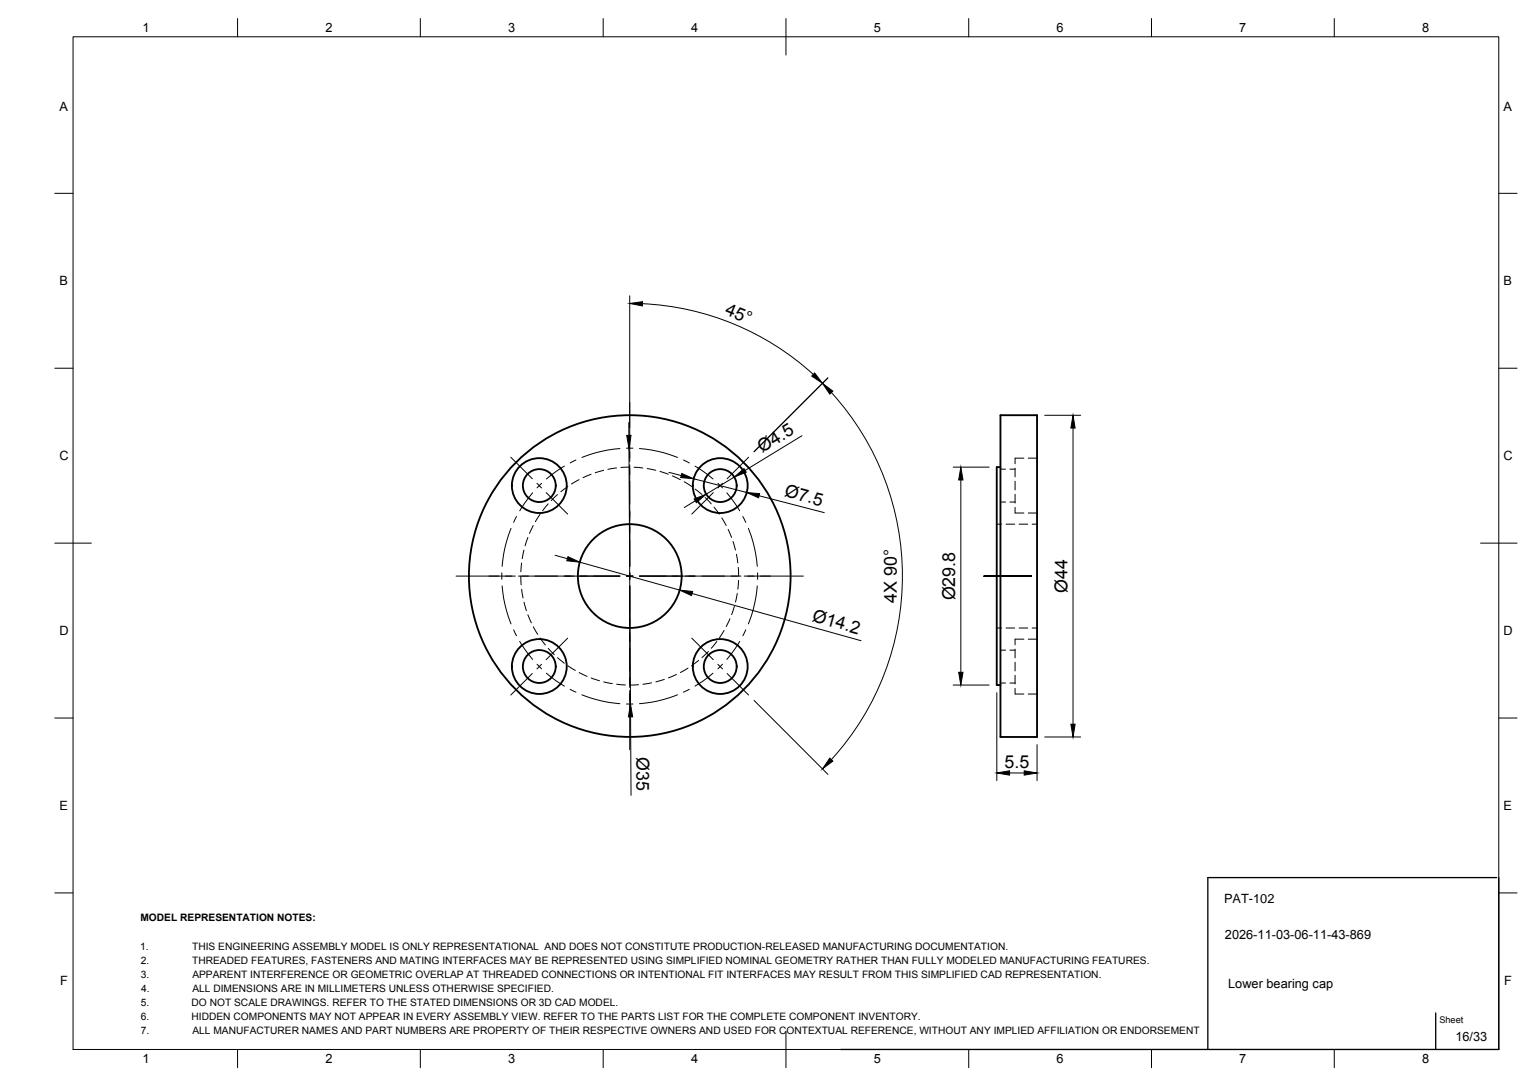
ISO-10303-21;
HEADER;
/* Generated by software containing ST-Developer
 * from STEP Tools, Inc. (www.steptools.com) 
 */

FILE_DESCRIPTION(
/* description */ ('Swing-away clamp arm'),
/* implementation_level */ '2;1');

FILE_NAME(
/* name */ 'Lower bearing cap.step',
/* time_stamp */ '2026-10-28T03:26:03-07:00',
/* author */ (''),
/* organization */ (''),
/* preprocessor_version */ 'ST-DEVELOPER v20.2',
/* originating_system */ 'Autodesk Translation Framework v15.17.0.0',
/* authorisation */ '');

FILE_SCHEMA (('AUTOMOTIVE_DESIGN { 1 0 10303 214 3 1 1 }'));
ENDSEC;

DATA;
#10=MECHANICAL_DESIGN_GEOMETRIC_PRESENTATION_REPRESENTATION('',(#303),#10627);
#251=SHAPE_REPRESENTATION_RELATIONSHIP('SRR','None',#10750,#277);
#277=ADVANCED_BREP_SHAPE_REPRESENTATION('',(#336),#10609);
#303=STYLED_ITEM('',(#10965),#336);
#336=MANIFOLD_SOLID_BREP('Body1',#4910);
#401=FACE_BOUND('',#1128,.T.);
#402=FACE_BOUND('',#1131,.T.);
#403=FACE_BOUND('',#1134,.T.);
#404=FACE_BOUND('',#1137,.T.);
#405=FACE_BOUND('',#1144,.T.);
#406=FACE_BOUND('',#1148,.T.);
#407=FACE_BOUND('',#1149,.T.);
#408=FACE_BOUND('',#1150,.T.);
#409=FACE_BOUND('',#1151,.T.);
#410=FACE_BOUND('',#1152,.T.);
#411=FACE_BOUND('',#1154,.T.);
#412=FACE_BOUND('',#1155,.T.);
#413=FACE_BOUND('',#1156,.T.);
#414=FACE_BOUND('',#1157,.T.);
#415=FACE_BOUND('',#1158,.T.);
#556=PLANE('',#5482);
#557=PLANE('',#5487);
#558=PLANE('',#5492);
#559=PLANE('',#5497);
#560=PLANE('',#5510);
#561=PLANE('',#5517);
#562=PLANE('',#5518);
#776=FACE_OUTER_BOUND('',#1126,.T.);
#777=FACE_OUTER_BOUND('',#1127,.T.);
#778=FACE_OUTER_BOUND('',#1129,.T.);
#779=FACE_OUTER_BOUND('',#1130,.T.);
#780=FACE_OUTER_BOUND('',#1132,.T.);
#781=FACE_OUTER_BOUND('',#1133,.T.);
#782=FACE_OUTER_BOUND('',#1135,.T.);
#783=FACE_OUTER_BOUND('',#1136,.T.);
#784=FACE_OUTER_BOUND('',#1138,.T.);
#785=FACE_OUTER_BOUND('',#1139,.T.);
#786=FACE_OUTER_BOUND('',#1140,.T.);
#787=FACE_OUTER_BOUND('',#1141,.T.);
#788=FACE_OUTER_BOUND('',#1142,.T.);
#789=FACE_OUTER_BOUND('',#1143,.T.);
#790=FACE_OUTER_BOUND('',#1145,.T.);
#791=FACE_OUTER_BOUND('',#1146,.T.);
#792=FACE_OUTER_BOUND('',#1147,.T.);
#793=FACE_OUTER_BOUND('',#1153,.T.);
#1126=EDGE_LOOP('',(#3873,#3874,#3875,#3876));
#1127=EDGE_LOOP('',(#3877));
#1128=EDGE_LOOP('',(#3878));
#1129=EDGE_LOOP('',(#3879,#3880,#3881,#3882));
#1130=EDGE_LOOP('',(#3883));
#1131=EDGE_LOOP('',(#3884));
#1132=EDGE_LOOP('',(#3885,#3886,#3887,#3888));
#1133=EDGE_LOOP('',(#3889));
#1134=EDGE_LOOP('',(#3890));
#1135=EDGE_LOOP('',(#3891,#3892,#3893,#3894));
#1136=EDGE_LOOP('',(#3895));
#1137=EDGE_LOOP('',(#3896));
#1138=EDGE_LOOP('',(#3897,#3898,#3899,#3900));
#1139=EDGE_LOOP('',(#3901,#3902,#3903,#3904));
#1140=EDGE_LOOP('',(#3905,#3906,#3907,#3908));
#1141=EDGE_LOOP('',(#3909,#3910,#3911,#3912));
#1142=EDGE_LOOP('',(#3913,#3914,#3915,#3916));
#1143=EDGE_LOOP('',(#3917));
#1144=EDGE_LOOP('',(#3918));
#1145=EDGE_LOOP('',(#3919,#3920,#3921,#3922));
#1146=EDGE_LOOP('',(#3923,#3924,#3925,#3926));
#1147=EDGE_LOOP('',(#3927));
#1148=EDGE_LOOP('',(#3928));
#1149=EDGE_LOOP('',(#3929));
#1150=EDGE_LOOP('',(#3930));
#1151=EDGE_LOOP('',(#3931));
#1152=EDGE_LOOP('',(#3932));
#1153=EDGE_LOOP('',(#3933));
#1154=EDGE_LOOP('',(#3934));
#1155=EDGE_LOOP('',(#3935));
#1156=EDGE_LOOP('',(#3936));
#1157=EDGE_LOOP('',(#3937));
#1158=EDGE_LOOP('',(#3938));
#1552=LINE('',#9485,#1874);
#1553=LINE('',#9494,#1875);
#1554=LINE('',#9503,#1876);
#1555=LINE('',#9512,#1877);
#1556=LINE('',#9519,#1878);
#1557=LINE('',#9523,#1879);
#1558=LINE('',#9527,#1880);
#1559=LINE('',#9531,#1881);
#1560=LINE('',#9537,#1882);
#1561=LINE('',#9544,#1883);
#1562=LINE('',#9550,#1884);
#1874=VECTOR('',#6587,0.375);
#1875=VECTOR('',#6598,0.375);
#1876=VECTOR('',#6609,0.375);
#1877=VECTOR('',#6620,0.375);
#1878=VECTOR('',#6629,0.225);
#1879=VECTOR('',#6634,0.225);
#1880=VECTOR('',#6639,0.225);
#1881=VECTOR('',#6644,0.225);
#1882=VECTOR('',#6651,1.49);
#1883=VECTOR('',#6660,0.71);
#1884=VECTOR('',#6667,2.2);
#2089=CIRCLE('',#5480,0.375);
#2090=CIRCLE('',#5481,0.375);
#2091=CIRCLE('',#5483,0.225);
#2092=CIRCLE('',#5485,0.375);
#2093=CIRCLE('',#5486,0.375);
#2094=CIRCLE('',#5488,0.225);
#2095=CIRCLE('',#5490,0.375);
#2096=CIRCLE('',#5491,0.375);
#2097=CIRCLE('',#5493,0.225);
#2098=CIRCLE('',#5495,0.375);
#2099=CIRCLE('',#5496,0.375);
#2100=CIRCLE('',#5498,0.225);
#2101=CIRCLE('',#5500,0.225);
#2102=CIRCLE('',#5502,0.225);
#2103=CIRCLE('',#5504,0.225);
#2104=CIRCLE('',#5506,0.225);
#2105=CIRCLE('',#5508,1.49);
#2106=CIRCLE('',#5509,1.49);
#2107=CIRCLE('',#5511,0.71);
#2108=CIRCLE('',#5513,0.71);
#2109=CIRCLE('',#5515,2.2);
#2110=CIRCLE('',#5516,2.2);
#2458=VERTEX_POINT('',#9482);
#2459=VERTEX_POINT('',#9484);
#2460=VERTEX_POINT('',#9488);
#2461=VERTEX_POINT('',#9491);
#2462=VERTEX_POINT('',#9493);
#2463=VERTEX_POINT('',#9497);
#2464=VERTEX_POINT('',#9500);
#2465=VERTEX_POINT('',#9502);
#2466=VERTEX_POINT('',#9506);
#2467=VERTEX_POINT('',#9509);
#2468=VERTEX_POINT('',#9511);
#2469=VERTEX_POINT('',#9515);
#2470=VERTEX_POINT('',#9518);
#2471=VERTEX_POINT('',#9522);
#2472=VERTEX_POINT('',#9526);
#2473=VERTEX_POINT('',#9530);
#2474=VERTEX_POINT('',#9534);
#2475=VERTEX_POINT('',#9536);
#2476=VERTEX_POINT('',#9540);
#2477=VERTEX_POINT('',#9543);
#2478=VERTEX_POINT('',#9547);
#2479=VERTEX_POINT('',#9549);
#2969=EDGE_CURVE('',#2458,#2458,#2089,.T.);
#2970=EDGE_CURVE('',#2458,#2459,#1552,.T.);
#2971=EDGE_CURVE('',#2459,#2459,#2090,.T.);
#2972=EDGE_CURVE('',#2460,#2460,#2091,.T.);
#2973=EDGE_CURVE('',#2461,#2461,#2092,.T.);
#2974=EDGE_CURVE('',#2461,#2462,#1553,.T.);
#2975=EDGE_CURVE('',#2462,#2462,#2093,.T.);
#2976=EDGE_CURVE('',#2463,#2463,#2094,.T.);
#2977=EDGE_CURVE('',#2464,#2464,#2095,.T.);
#2978=EDGE_CURVE('',#2464,#2465,#1554,.T.);
#2979=EDGE_CURVE('',#2465,#2465,#2096,.T.);
#2980=EDGE_CURVE('',#2466,#2466,#2097,.T.);
#2981=EDGE_CURVE('',#2467,#2467,#2098,.T.);
#2982=EDGE_CURVE('',#2467,#2468,#1555,.T.);
#2983=EDGE_CURVE('',#2468,#2468,#2099,.T.);
#2984=EDGE_CURVE('',#2469,#2469,#2100,.T.);
#2985=EDGE_CURVE('',#2460,#2470,#1556,.T.);
#2986=EDGE_CURVE('',#2470,#2470,#2101,.T.);
#2987=EDGE_CURVE('',#2463,#2471,#1557,.T.);
#2988=EDGE_CURVE('',#2471,#2471,#2102,.T.);
#2989=EDGE_CURVE('',#2466,#2472,#1558,.T.);
#2990=EDGE_CURVE('',#2472,#2472,#2103,.T.);
#2991=EDGE_CURVE('',#2469,#2473,#1559,.T.);
#2992=EDGE_CURVE('',#2473,#2473,#2104,.T.);
#2993=EDGE_CURVE('',#2474,#2474,#2105,.T.);
#2994=EDGE_CURVE('',#2474,#2475,#1560,.T.);
#2995=EDGE_CURVE('',#2475,#2475,#2106,.T.);
#2996=EDGE_CURVE('',#2476,#2476,#2107,.T.);
#2997=EDGE_CURVE('',#2476,#2477,#1561,.T.);
#2998=EDGE_CURVE('',#2477,#2477,#2108,.T.);
#2999=EDGE_CURVE('',#2478,#2478,#2109,.T.);
#3000=EDGE_CURVE('',#2478,#2479,#1562,.T.);
#3001=EDGE_CURVE('',#2479,#2479,#2110,.T.);
#3873=ORIENTED_EDGE('',*,*,#2969,.F.);
#3874=ORIENTED_EDGE('',*,*,#2970,.T.);
#3875=ORIENTED_EDGE('',*,*,#2971,.T.);
#3876=ORIENTED_EDGE('',*,*,#2970,.F.);
#3877=ORIENTED_EDGE('',*,*,#2971,.F.);
#3878=ORIENTED_EDGE('',*,*,#2972,.F.);
#3879=ORIENTED_EDGE('',*,*,#2973,.F.);
#3880=ORIENTED_EDGE('',*,*,#2974,.T.);
#3881=ORIENTED_EDGE('',*,*,#2975,.T.);
#3882=ORIENTED_EDGE('',*,*,#2974,.F.);
#3883=ORIENTED_EDGE('',*,*,#2975,.F.);
#3884=ORIENTED_EDGE('',*,*,#2976,.F.);
#3885=ORIENTED_EDGE('',*,*,#2977,.F.);
#3886=ORIENTED_EDGE('',*,*,#2978,.T.);
#3887=ORIENTED_EDGE('',*,*,#2979,.T.);
#3888=ORIENTED_EDGE('',*,*,#2978,.F.);
#3889=ORIENTED_EDGE('',*,*,#2979,.F.);
#3890=ORIENTED_EDGE('',*,*,#2980,.F.);
#3891=ORIENTED_EDGE('',*,*,#2981,.F.);
#3892=ORIENTED_EDGE('',*,*,#2982,.T.);
#3893=ORIENTED_EDGE('',*,*,#2983,.T.);
#3894=ORIENTED_EDGE('',*,*,#2982,.F.);
#3895=ORIENTED_EDGE('',*,*,#2983,.F.);
#3896=ORIENTED_EDGE('',*,*,#2984,.F.);
#3897=ORIENTED_EDGE('',*,*,#2972,.T.);
#3898=ORIENTED_EDGE('',*,*,#2985,.T.);
#3899=ORIENTED_EDGE('',*,*,#2986,.F.);
#3900=ORIENTED_EDGE('',*,*,#2985,.F.);
#3901=ORIENTED_EDGE('',*,*,#2976,.T.);
#3902=ORIENTED_EDGE('',*,*,#2987,.T.);
#3903=ORIENTED_EDGE('',*,*,#2988,.F.);
#3904=ORIENTED_EDGE('',*,*,#2987,.F.);
#3905=ORIENTED_EDGE('',*,*,#2980,.T.);
#3906=ORIENTED_EDGE('',*,*,#2989,.T.);
#3907=ORIENTED_EDGE('',*,*,#2990,.F.);
#3908=ORIENTED_EDGE('',*,*,#2989,.F.);
#3909=ORIENTED_EDGE('',*,*,#2984,.T.);
#3910=ORIENTED_EDGE('',*,*,#2991,.T.);
#3911=ORIENTED_EDGE('',*,*,#2992,.F.);
#3912=ORIENTED_EDGE('',*,*,#2991,.F.);
#3913=ORIENTED_EDGE('',*,*,#2993,.F.);
#3914=ORIENTED_EDGE('',*,*,#2994,.T.);
#3915=ORIENTED_EDGE('',*,*,#2995,.F.);
#3916=ORIENTED_EDGE('',*,*,#2994,.F.);
#3917=ORIENTED_EDGE('',*,*,#2993,.T.);
#3918=ORIENTED_EDGE('',*,*,#2996,.T.);
#3919=ORIENTED_EDGE('',*,*,#2996,.F.);
#3920=ORIENTED_EDGE('',*,*,#2997,.T.);
#3921=ORIENTED_EDGE('',*,*,#2998,.T.);
#3922=ORIENTED_EDGE('',*,*,#2997,.F.);
#3923=ORIENTED_EDGE('',*,*,#2999,.F.);
#3924=ORIENTED_EDGE('',*,*,#3000,.T.);
#3925=ORIENTED_EDGE('',*,*,#3001,.T.);
#3926=ORIENTED_EDGE('',*,*,#3000,.F.);
#3927=ORIENTED_EDGE('',*,*,#2999,.T.);
#3928=ORIENTED_EDGE('',*,*,#2995,.T.);
#3929=ORIENTED_EDGE('',*,*,#2992,.T.);
#3930=ORIENTED_EDGE('',*,*,#2990,.T.);
#3931=ORIENTED_EDGE('',*,*,#2988,.T.);
#3932=ORIENTED_EDGE('',*,*,#2986,.T.);
#3933=ORIENTED_EDGE('',*,*,#3001,.F.);
#3934=ORIENTED_EDGE('',*,*,#2998,.F.);
#3935=ORIENTED_EDGE('',*,*,#2981,.T.);
#3936=ORIENTED_EDGE('',*,*,#2977,.T.);
#3937=ORIENTED_EDGE('',*,*,#2973,.T.);
#3938=ORIENTED_EDGE('',*,*,#2969,.T.);
#4534=CYLINDRICAL_SURFACE('',#5479,0.375);
#4535=CYLINDRICAL_SURFACE('',#5484,0.375);
#4536=CYLINDRICAL_SURFACE('',#5489,0.375);
#4537=CYLINDRICAL_SURFACE('',#5494,0.375);
#4538=CYLINDRICAL_SURFACE('',#5499,0.225);
#4539=CYLINDRICAL_SURFACE('',#5501,0.225);
#4540=CYLINDRICAL_SURFACE('',#5503,0.225);
#4541=CYLINDRICAL_SURFACE('',#5505,0.225);
#4542=CYLINDRICAL_SURFACE('',#5507,1.49);
#4543=CYLINDRICAL_SURFACE('',#5512,0.71);
#4544=CYLINDRICAL_SURFACE('',#5514,2.2);
#4731=ADVANCED_FACE('',(#776),#4534,.F.);
#4732=ADVANCED_FACE('',(#777,#401),#556,.F.);
#4733=ADVANCED_FACE('',(#778),#4535,.F.);
#4734=ADVANCED_FACE('',(#779,#402),#557,.F.);
#4735=ADVANCED_FACE('',(#780),#4536,.F.);
#4736=ADVANCED_FACE('',(#781,#403),#558,.F.);
#4737=ADVANCED_FACE('',(#782),#4537,.F.);
#4738=ADVANCED_FACE('',(#783,#404),#559,.F.);
#4739=ADVANCED_FACE('',(#784),#4538,.F.);
#4740=ADVANCED_FACE('',(#785),#4539,.F.);
#4741=ADVANCED_FACE('',(#786),#4540,.F.);
#4742=ADVANCED_FACE('',(#787),#4541,.F.);
#4743=ADVANCED_FACE('',(#788),#4542,.T.);
#4744=ADVANCED_FACE('',(#789,#405),#560,.T.);
#4745=ADVANCED_FACE('',(#790),#4543,.F.);
#4746=ADVANCED_FACE('',(#791),#4544,.T.);
#4747=ADVANCED_FACE('',(#792,#406,#407,#408,#409,#410),#561,.T.);
#4748=ADVANCED_FACE('',(#793,#411,#412,#413,#414,#415),#562,.F.);
#4910=CLOSED_SHELL('',(#4731,#4732,#4733,#4734,#4735,#4736,#4737,#4738,
#4739,#4740,#4741,#4742,#4743,#4744,#4745,#4746,#4747,#4748));
#5478=AXIS2_PLACEMENT_3D('',#9480,#6581,#6582);
#5479=AXIS2_PLACEMENT_3D('',#9481,#6583,#6584);
#5480=AXIS2_PLACEMENT_3D('',#9483,#6585,#6586);
#5481=AXIS2_PLACEMENT_3D('',#9486,#6588,#6589);
#5482=AXIS2_PLACEMENT_3D('',#9487,#6590,#6591);
#5483=AXIS2_PLACEMENT_3D('',#9489,#6592,#6593);
#5484=AXIS2_PLACEMENT_3D('',#9490,#6594,#6595);
#5485=AXIS2_PLACEMENT_3D('',#9492,#6596,#6597);
#5486=AXIS2_PLACEMENT_3D('',#9495,#6599,#6600);
#5487=AXIS2_PLACEMENT_3D('',#9496,#6601,#6602);
#5488=AXIS2_PLACEMENT_3D('',#9498,#6603,#6604);
#5489=AXIS2_PLACEMENT_3D('',#9499,#6605,#6606);
#5490=AXIS2_PLACEMENT_3D('',#9501,#6607,#6608);
#5491=AXIS2_PLACEMENT_3D('',#9504,#6610,#6611);
#5492=AXIS2_PLACEMENT_3D('',#9505,#6612,#6613);
#5493=AXIS2_PLACEMENT_3D('',#9507,#6614,#6615);
#5494=AXIS2_PLACEMENT_3D('',#9508,#6616,#6617);
#5495=AXIS2_PLACEMENT_3D('',#9510,#6618,#6619);
#5496=AXIS2_PLACEMENT_3D('',#9513,#6621,#6622);
#5497=AXIS2_PLACEMENT_3D('',#9514,#6623,#6624);
#5498=AXIS2_PLACEMENT_3D('',#9516,#6625,#6626);
#5499=AXIS2_PLACEMENT_3D('',#9517,#6627,#6628);
#5500=AXIS2_PLACEMENT_3D('',#9520,#6630,#6631);
#5501=AXIS2_PLACEMENT_3D('',#9521,#6632,#6633);
#5502=AXIS2_PLACEMENT_3D('',#9524,#6635,#6636);
#5503=AXIS2_PLACEMENT_3D('',#9525,#6637,#6638);
#5504=AXIS2_PLACEMENT_3D('',#9528,#6640,#6641);
#5505=AXIS2_PLACEMENT_3D('',#9529,#6642,#6643);
#5506=AXIS2_PLACEMENT_3D('',#9532,#6645,#6646);
#5507=AXIS2_PLACEMENT_3D('',#9533,#6647,#6648);
#5508=AXIS2_PLACEMENT_3D('',#9535,#6649,#6650);
#5509=AXIS2_PLACEMENT_3D('',#9538,#6652,#6653);
#5510=AXIS2_PLACEMENT_3D('',#9539,#6654,#6655);
#5511=AXIS2_PLACEMENT_3D('',#9541,#6656,#6657);
#5512=AXIS2_PLACEMENT_3D('',#9542,#6658,#6659);
#5513=AXIS2_PLACEMENT_3D('',#9545,#6661,#6662);
#5514=AXIS2_PLACEMENT_3D('',#9546,#6663,#6664);
#5515=AXIS2_PLACEMENT_3D('',#9548,#6665,#6666);
#5516=AXIS2_PLACEMENT_3D('',#9551,#6668,#6669);
#5517=AXIS2_PLACEMENT_3D('',#9552,#6670,#6671);
#5518=AXIS2_PLACEMENT_3D('',#9553,#6672,#6673);
#6581=DIRECTION('axis',(0.,0.,1.));
#6582=DIRECTION('refdir',(1.,0.,0.));
#6583=DIRECTION('center_axis',(0.,0.,1.));
#6584=DIRECTION('ref_axis',(1.,0.,0.));
#6585=DIRECTION('center_axis',(0.,0.,1.));
#6586=DIRECTION('ref_axis',(1.,0.,0.));
#6587=DIRECTION('',(0.,0.,1.));
#6588=DIRECTION('center_axis',(0.,0.,1.));
#6589=DIRECTION('ref_axis',(1.,0.,0.));
#6590=DIRECTION('center_axis',(0.,0.,1.));
#6591=DIRECTION('ref_axis',(1.,0.,0.));
#6592=DIRECTION('center_axis',(0.,0.,-1.));
#6593=DIRECTION('ref_axis',(1.,0.,0.));
#6594=DIRECTION('center_axis',(0.,0.,1.));
#6595=DIRECTION('ref_axis',(1.,0.,0.));
#6596=DIRECTION('center_axis',(0.,0.,1.));
#6597=DIRECTION('ref_axis',(1.,0.,0.));
#6598=DIRECTION('',(0.,0.,1.));
#6599=DIRECTION('center_axis',(0.,0.,1.));
#6600=DIRECTION('ref_axis',(1.,0.,0.));
#6601=DIRECTION('center_axis',(0.,0.,1.));
#6602=DIRECTION('ref_axis',(1.,0.,0.));
#6603=DIRECTION('center_axis',(0.,0.,-1.));
#6604=DIRECTION('ref_axis',(1.,0.,0.));
#6605=DIRECTION('center_axis',(0.,0.,1.));
#6606=DIRECTION('ref_axis',(1.,0.,0.));
#6607=DIRECTION('center_axis',(0.,0.,1.));
#6608=DIRECTION('ref_axis',(1.,0.,0.));
#6609=DIRECTION('',(0.,0.,1.));
#6610=DIRECTION('center_axis',(0.,0.,1.));
#6611=DIRECTION('ref_axis',(1.,0.,0.));
#6612=DIRECTION('center_axis',(0.,0.,1.));
#6613=DIRECTION('ref_axis',(1.,0.,0.));
#6614=DIRECTION('center_axis',(0.,0.,-1.));
#6615=DIRECTION('ref_axis',(1.,0.,0.));
#6616=DIRECTION('center_axis',(0.,0.,1.));
#6617=DIRECTION('ref_axis',(1.,0.,0.));
#6618=DIRECTION('center_axis',(0.,0.,1.));
#6619=DIRECTION('ref_axis',(1.,0.,0.));
#6620=DIRECTION('',(0.,0.,1.));
#6621=DIRECTION('center_axis',(0.,0.,1.));
#6622=DIRECTION('ref_axis',(1.,0.,0.));
#6623=DIRECTION('center_axis',(0.,0.,1.));
#6624=DIRECTION('ref_axis',(1.,0.,0.));
#6625=DIRECTION('center_axis',(0.,0.,-1.));
#6626=DIRECTION('ref_axis',(1.,0.,0.));
#6627=DIRECTION('center_axis',(0.,0.,1.));
#6628=DIRECTION('ref_axis',(1.,0.,0.));
#6629=DIRECTION('',(0.,0.,1.));
#6630=DIRECTION('center_axis',(0.,0.,-1.));
#6631=DIRECTION('ref_axis',(1.,0.,0.));
#6632=DIRECTION('center_axis',(0.,0.,1.));
#6633=DIRECTION('ref_axis',(1.,0.,0.));
#6634=DIRECTION('',(0.,0.,1.));
#6635=DIRECTION('center_axis',(0.,0.,-1.));
#6636=DIRECTION('ref_axis',(1.,0.,0.));
#6637=DIRECTION('center_axis',(0.,0.,1.));
#6638=DIRECTION('ref_axis',(1.,0.,0.));
#6639=DIRECTION('',(0.,0.,1.));
#6640=DIRECTION('center_axis',(0.,0.,-1.));
#6641=DIRECTION('ref_axis',(1.,0.,0.));
#6642=DIRECTION('center_axis',(0.,0.,1.));
#6643=DIRECTION('ref_axis',(1.,0.,0.));
#6644=DIRECTION('',(0.,0.,1.));
#6645=DIRECTION('center_axis',(0.,0.,-1.));
#6646=DIRECTION('ref_axis',(1.,0.,0.));
#6647=DIRECTION('center_axis',(0.,0.,1.));
#6648=DIRECTION('ref_axis',(1.,0.,0.));
#6649=DIRECTION('center_axis',(0.,0.,1.));
#6650=DIRECTION('ref_axis',(1.,0.,0.));
#6651=DIRECTION('',(0.,0.,-1.));
#6652=DIRECTION('center_axis',(0.,0.,-1.));
#6653=DIRECTION('ref_axis',(1.,0.,0.));
#6654=DIRECTION('center_axis',(0.,0.,1.));
#6655=DIRECTION('ref_axis',(1.,0.,0.));
#6656=DIRECTION('center_axis',(0.,0.,-1.));
#6657=DIRECTION('ref_axis',(1.,0.,0.));
#6658=DIRECTION('center_axis',(0.,0.,1.));
#6659=DIRECTION('ref_axis',(1.,0.,0.));
#6660=DIRECTION('',(0.,0.,-1.));
#6661=DIRECTION('center_axis',(0.,0.,-1.));
#6662=DIRECTION('ref_axis',(1.,0.,0.));
#6663=DIRECTION('center_axis',(0.,0.,1.));
#6664=DIRECTION('ref_axis',(1.,0.,0.));
#6665=DIRECTION('center_axis',(0.,0.,1.));
#6666=DIRECTION('ref_axis',(1.,0.,0.));
#6667=DIRECTION('',(0.,0.,-1.));
#6668=DIRECTION('center_axis',(0.,0.,1.));
#6669=DIRECTION('ref_axis',(1.,0.,0.));
#6670=DIRECTION('center_axis',(0.,0.,1.));
#6671=DIRECTION('ref_axis',(1.,0.,0.));
#6672=DIRECTION('center_axis',(0.,0.,1.));
#6673=DIRECTION('ref_axis',(1.,0.,0.));
#9480=CARTESIAN_POINT('',(0.,0.,0.));
#9481=CARTESIAN_POINT('Origin',(-1.23743686707646,-1.23743686707646,5.4));
#9482=CARTESIAN_POINT('',(-1.61243686707646,-1.23743686707646,5.5));
#9483=CARTESIAN_POINT('Origin',(-1.23743686707646,-1.23743686707646,5.5));
#9484=CARTESIAN_POINT('',(-1.61243686707646,-1.23743686707646,5.8));
#9485=CARTESIAN_POINT('',(-1.61243686707646,-1.23743686707646,5.4));
#9486=CARTESIAN_POINT('Origin',(-1.23743686707646,-1.23743686707646,5.8));
#9487=CARTESIAN_POINT('Origin',(-1.23743686707646,-1.23743686707646,5.8));
#9488=CARTESIAN_POINT('',(-1.46243686707646,-1.23743686707646,5.8));
#9489=CARTESIAN_POINT('Origin',(-1.23743686707646,-1.23743686707646,5.8));
#9490=CARTESIAN_POINT('Origin',(-1.23743686707646,1.23743686707646,5.4));
#9491=CARTESIAN_POINT('',(-1.61243686707646,1.23743686707646,5.5));
#9492=CARTESIAN_POINT('Origin',(-1.23743686707646,1.23743686707646,5.5));
#9493=CARTESIAN_POINT('',(-1.61243686707646,1.23743686707646,5.8));
#9494=CARTESIAN_POINT('',(-1.61243686707646,1.23743686707646,5.4));
#9495=CARTESIAN_POINT('Origin',(-1.23743686707646,1.23743686707646,5.8));
#9496=CARTESIAN_POINT('Origin',(-1.23743686707646,1.23743686707646,5.8));
#9497=CARTESIAN_POINT('',(-1.46243686707646,1.23743686707646,5.8));
#9498=CARTESIAN_POINT('Origin',(-1.23743686707646,1.23743686707646,5.8));
#9499=CARTESIAN_POINT('Origin',(1.23743686707646,1.23743686707646,5.4));
#9500=CARTESIAN_POINT('',(0.862436867076458,1.23743686707646,5.5));
#9501=CARTESIAN_POINT('Origin',(1.23743686707646,1.23743686707646,5.5));
#9502=CARTESIAN_POINT('',(0.862436867076458,1.23743686707646,5.8));
#9503=CARTESIAN_POINT('',(0.862436867076458,1.23743686707646,5.4));
#9504=CARTESIAN_POINT('Origin',(1.23743686707646,1.23743686707646,5.8));
#9505=CARTESIAN_POINT('Origin',(1.23743686707646,1.23743686707646,5.8));
#9506=CARTESIAN_POINT('',(1.01243686707646,1.23743686707646,5.8));
#9507=CARTESIAN_POINT('Origin',(1.23743686707646,1.23743686707646,5.8));
#9508=CARTESIAN_POINT('Origin',(1.23743686707646,-1.23743686707646,5.4));
#9509=CARTESIAN_POINT('',(0.862436867076458,-1.23743686707646,5.5));
#9510=CARTESIAN_POINT('Origin',(1.23743686707646,-1.23743686707646,5.5));
#9511=CARTESIAN_POINT('',(0.862436867076458,-1.23743686707646,5.8));
#9512=CARTESIAN_POINT('',(0.862436867076458,-1.23743686707646,5.4));
#9513=CARTESIAN_POINT('Origin',(1.23743686707646,-1.23743686707646,5.8));
#9514=CARTESIAN_POINT('Origin',(1.23743686707646,-1.23743686707646,5.8));
#9515=CARTESIAN_POINT('',(1.01243686707646,-1.23743686707646,5.8));
#9516=CARTESIAN_POINT('Origin',(1.23743686707646,-1.23743686707646,5.8));
#9517=CARTESIAN_POINT('Origin',(-1.23743686707646,-1.23743686707646,5.4));
#9518=CARTESIAN_POINT('',(-1.46243686707646,-1.23743686707646,6.));
#9519=CARTESIAN_POINT('',(-1.46243686707646,-1.23743686707646,5.4));
#9520=CARTESIAN_POINT('Origin',(-1.23743686707646,-1.23743686707646,6.));
#9521=CARTESIAN_POINT('Origin',(-1.23743686707646,1.23743686707646,5.4));
#9522=CARTESIAN_POINT('',(-1.46243686707646,1.23743686707646,6.));
#9523=CARTESIAN_POINT('',(-1.46243686707646,1.23743686707646,5.4));
#9524=CARTESIAN_POINT('Origin',(-1.23743686707646,1.23743686707646,6.));
#9525=CARTESIAN_POINT('Origin',(1.23743686707646,1.23743686707646,5.4));
#9526=CARTESIAN_POINT('',(1.01243686707646,1.23743686707646,6.));
#9527=CARTESIAN_POINT('',(1.01243686707646,1.23743686707646,5.4));
#9528=CARTESIAN_POINT('Origin',(1.23743686707646,1.23743686707646,6.));
#9529=CARTESIAN_POINT('Origin',(1.23743686707646,-1.23743686707646,5.4));
#9530=CARTESIAN_POINT('',(1.01243686707646,-1.23743686707646,6.));
#9531=CARTESIAN_POINT('',(1.01243686707646,-1.23743686707646,5.4));
#9532=CARTESIAN_POINT('Origin',(1.23743686707646,-1.23743686707646,6.));
#9533=CARTESIAN_POINT('Origin',(0.,0.,6.));
#9534=CARTESIAN_POINT('',(-1.49,-1.82472373072956E-16,6.05));
#9535=CARTESIAN_POINT('Origin',(0.,0.,6.05));
#9536=CARTESIAN_POINT('',(-1.49,-1.82472373072956E-16,6.));
#9537=CARTESIAN_POINT('',(-1.49,-1.82472373072956E-16,6.));
#9538=CARTESIAN_POINT('Origin',(0.,0.,6.));
#9539=CARTESIAN_POINT('Origin',(0.,0.,6.05));
#9540=CARTESIAN_POINT('',(-0.71,-8.69499227394621E-17,6.05));
#9541=CARTESIAN_POINT('Origin',(0.,0.,6.05));
#9542=CARTESIAN_POINT('Origin',(0.,0.,5.5));
#9543=CARTESIAN_POINT('',(-0.71,-8.69499227394621E-17,5.5));
#9544=CARTESIAN_POINT('',(-0.71,-8.69499227394621E-17,5.5));
#9545=CARTESIAN_POINT('Origin',(0.,0.,5.5));
#9546=CARTESIAN_POINT('Origin',(0.,0.,5.5));
#9547=CARTESIAN_POINT('',(-2.2,-2.69422295812418E-16,6.));
#9548=CARTESIAN_POINT('Origin',(0.,0.,6.));
#9549=CARTESIAN_POINT('',(-2.2,-2.69422295812418E-16,5.5));
#9550=CARTESIAN_POINT('',(-2.2,-2.69422295812418E-16,5.5));
#9551=CARTESIAN_POINT('Origin',(0.,0.,5.5));
#9552=CARTESIAN_POINT('Origin',(0.,0.,6.));
#9553=CARTESIAN_POINT('Origin',(0.,0.,5.5));
#10577=UNCERTAINTY_MEASURE_WITH_UNIT(LENGTH_MEASURE(0.001),#10628,
'DISTANCE_ACCURACY_VALUE',
'Maximum model space distance between geometric entities at asserted c
onnectivities');
#10595=UNCERTAINTY_MEASURE_WITH_UNIT(LENGTH_MEASURE(0.001),#10628,
'DISTANCE_ACCURACY_VALUE',
'Maximum model space distance between geometric entities at asserted c
onnectivities');
#10609=(
GEOMETRIC_REPRESENTATION_CONTEXT(3)
GLOBAL_UNCERTAINTY_ASSIGNED_CONTEXT((#10577))
GLOBAL_UNIT_ASSIGNED_CONTEXT((#10628,#10630,#10631))
REPRESENTATION_CONTEXT('','3D')
);
#10627=(
GEOMETRIC_REPRESENTATION_CONTEXT(3)
GLOBAL_UNCERTAINTY_ASSIGNED_CONTEXT((#10595))
GLOBAL_UNIT_ASSIGNED_CONTEXT((#10628,#10630,#10631))
REPRESENTATION_CONTEXT('','3D')
);
#10628=(
LENGTH_UNIT()
NAMED_UNIT(*)
SI_UNIT(.CENTI.,.METRE.)
);
#10630=(
NAMED_UNIT(*)
PLANE_ANGLE_UNIT()
SI_UNIT($,.RADIAN.)
);
#10631=(
NAMED_UNIT(*)
SI_UNIT($,.STERADIAN.)
SOLID_ANGLE_UNIT()
);
#10645=SHAPE_DEFINITION_REPRESENTATION(#10686,#10750);
#10686=PRODUCT_DEFINITION_SHAPE('',$,#10782);
#10750=SHAPE_REPRESENTATION('',(#5478),#10609);
#10768=PRODUCT_DEFINITION_CONTEXT('part definition',#10863,'design');
#10782=PRODUCT_DEFINITION('Lower bearing cap','Lower bearing cap',#10813,
#10768);
#10813=PRODUCT_DEFINITION_FORMATION('',$,#10878);
#10863=APPLICATION_CONTEXT(
'Core Data for Automotive Mechanical Design Process');
#10864=PRODUCT_CONTEXT('part definition',#10863,'mechanical');
#10878=PRODUCT('Lower bearing cap','Lower bearing cap',
'Lower bearing cap',(#10864));
#10959=COLOUR_RGB('Grey',0.48,0.52,0.57);
#10960=FILL_AREA_STYLE_COLOUR('',#10959);
#10961=FILL_AREA_STYLE('',(#10960));
#10962=SURFACE_STYLE_FILL_AREA(#10961);
#10963=SURFACE_SIDE_STYLE('',(#10962));
#10964=SURFACE_STYLE_USAGE(.BOTH.,#10963);
#10965=PRESENTATION_STYLE_ASSIGNMENT((#10964));
ENDSEC;
END-ISO-10303-21;
